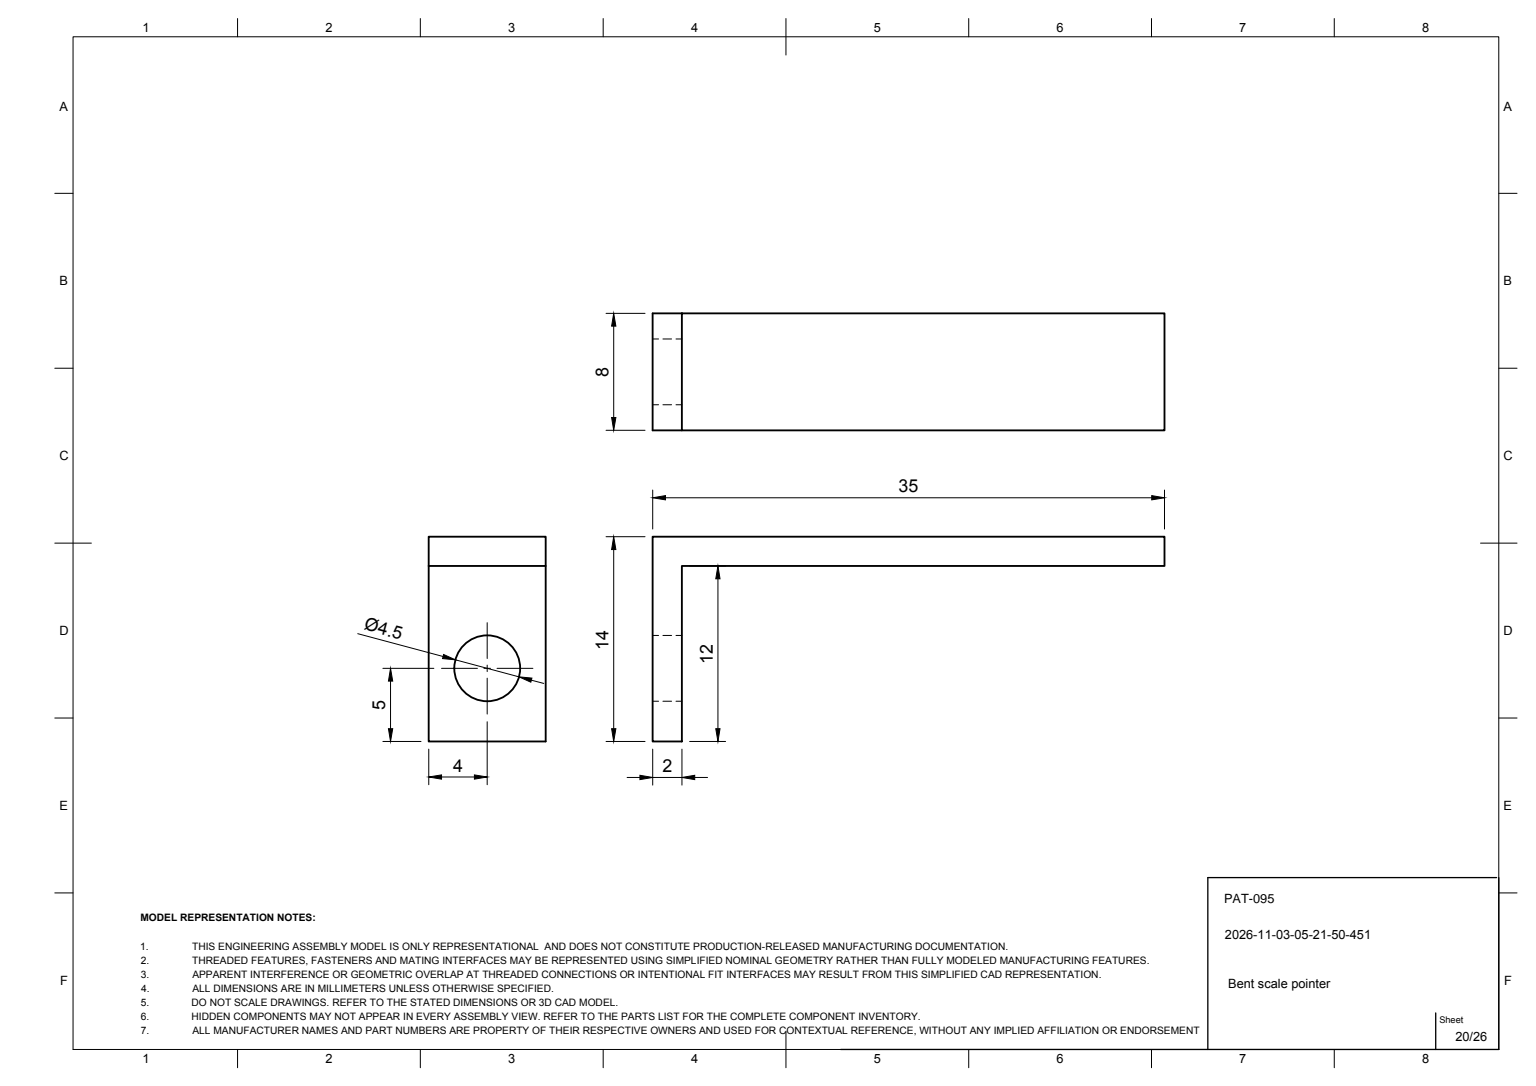
ISO-10303-21;
HEADER;
/* Generated by software containing ST-Developer
 * from STEP Tools, Inc. (www.steptools.com) 
 */

FILE_DESCRIPTION(
/* description */ ('Single-Axis Profile-Rail Linear Slide'),
/* implementation_level */ '2;1');

FILE_NAME(
/* name */ 'Bent scale pointer.step',
/* time_stamp */ '2026-10-27T10:47:43-07:00',
/* author */ (''),
/* organization */ (''),
/* preprocessor_version */ 'ST-DEVELOPER v20.2',
/* originating_system */ 'Autodesk Translation Framework v15.17.0.0',
/* authorisation */ '');

FILE_SCHEMA (('AUTOMOTIVE_DESIGN { 1 0 10303 214 3 1 1 }'));
ENDSEC;

DATA;
#10=MECHANICAL_DESIGN_GEOMETRIC_PRESENTATION_REPRESENTATION('',(#345),#14478);
#291=SHAPE_REPRESENTATION_RELATIONSHIP('SRR','None',#14622,#318);
#318=ADVANCED_BREP_SHAPE_REPRESENTATION('',(#370),#14466);
#345=STYLED_ITEM('',(#14845),#370);
#370=MANIFOLD_SOLID_BREP('Body1',#8607);
#451=FACE_BOUND('',#1705,.T.);
#452=FACE_BOUND('',#1710,.T.);
#753=PLANE('',#9375);
#754=PLANE('',#9376);
#755=PLANE('',#9377);
#756=PLANE('',#9378);
#757=PLANE('',#9379);
#758=PLANE('',#9380);
#759=PLANE('',#9381);
#760=PLANE('',#9382);
#1175=FACE_OUTER_BOUND('',#1703,.T.);
#1176=FACE_OUTER_BOUND('',#1704,.T.);
#1177=FACE_OUTER_BOUND('',#1706,.T.);
#1178=FACE_OUTER_BOUND('',#1707,.T.);
#1179=FACE_OUTER_BOUND('',#1708,.T.);
#1180=FACE_OUTER_BOUND('',#1709,.T.);
#1181=FACE_OUTER_BOUND('',#1711,.T.);
#1182=FACE_OUTER_BOUND('',#1712,.T.);
#1183=FACE_OUTER_BOUND('',#1713,.T.);
#1703=EDGE_LOOP('',(#7541,#7542,#7543,#7544));
#1704=EDGE_LOOP('',(#7545,#7546,#7547,#7548));
#1705=EDGE_LOOP('',(#7549));
#1706=EDGE_LOOP('',(#7550,#7551,#7552,#7553));
#1707=EDGE_LOOP('',(#7554,#7555,#7556,#7557));
#1708=EDGE_LOOP('',(#7558,#7559,#7560,#7561));
#1709=EDGE_LOOP('',(#7562,#7563,#7564,#7565));
#1710=EDGE_LOOP('',(#7566));
#1711=EDGE_LOOP('',(#7567,#7568,#7569,#7570));
#1712=EDGE_LOOP('',(#7571,#7572,#7573,#7574,#7575,#7576));
#1713=EDGE_LOOP('',(#7577,#7578,#7579,#7580,#7581,#7582));
#2606=LINE('',#13793,#3577);
#2607=LINE('',#13798,#3578);
#2608=LINE('',#13800,#3579);
#2609=LINE('',#13802,#3580);
#2610=LINE('',#13803,#3581);
#2611=LINE('',#13806,#3582);
#2612=LINE('',#13808,#3583);
#2613=LINE('',#13809,#3584);
#2614=LINE('',#13812,#3585);
#2615=LINE('',#13814,#3586);
#2616=LINE('',#13815,#3587);
#2617=LINE('',#13818,#3588);
#2618=LINE('',#13820,#3589);
#2619=LINE('',#13821,#3590);
#2620=LINE('',#13824,#3591);
#2621=LINE('',#13826,#3592);
#2622=LINE('',#13827,#3593);
#2623=LINE('',#13829,#3594);
#2624=LINE('',#13830,#3595);
#3577=VECTOR('',#11297,0.225);
#3578=VECTOR('',#11302,1.);
#3579=VECTOR('',#11303,1.);
#3580=VECTOR('',#11304,1.);
#3581=VECTOR('',#11305,1.);
#3582=VECTOR('',#11308,1.);
#3583=VECTOR('',#11309,1.);
#3584=VECTOR('',#11310,1.);
#3585=VECTOR('',#11313,1.);
#3586=VECTOR('',#11314,1.);
#3587=VECTOR('',#11315,1.);
#3588=VECTOR('',#11318,1.);
#3589=VECTOR('',#11319,1.);
#3590=VECTOR('',#11320,1.);
#3591=VECTOR('',#11323,1.);
#3592=VECTOR('',#11324,1.);
#3593=VECTOR('',#11325,1.);
#3594=VECTOR('',#11328,1.);
#3595=VECTOR('',#11329,1.);
#3878=CIRCLE('',#9373,0.225);
#3879=CIRCLE('',#9374,0.225);
#4512=VERTEX_POINT('',#13790);
#4513=VERTEX_POINT('',#13792);
#4514=VERTEX_POINT('',#13796);
#4515=VERTEX_POINT('',#13797);
#4516=VERTEX_POINT('',#13799);
#4517=VERTEX_POINT('',#13801);
#4518=VERTEX_POINT('',#13805);
#4519=VERTEX_POINT('',#13807);
#4520=VERTEX_POINT('',#13811);
#4521=VERTEX_POINT('',#13813);
#4522=VERTEX_POINT('',#13817);
#4523=VERTEX_POINT('',#13819);
#4524=VERTEX_POINT('',#13823);
#4525=VERTEX_POINT('',#13825);
#5548=EDGE_CURVE('',#4512,#4512,#3878,.T.);
#5549=EDGE_CURVE('',#4512,#4513,#2606,.T.);
#5550=EDGE_CURVE('',#4513,#4513,#3879,.T.);
#5551=EDGE_CURVE('',#4514,#4515,#2607,.T.);
#5552=EDGE_CURVE('',#4515,#4516,#2608,.T.);
#5553=EDGE_CURVE('',#4517,#4516,#2609,.T.);
#5554=EDGE_CURVE('',#4514,#4517,#2610,.T.);
#5555=EDGE_CURVE('',#4518,#4514,#2611,.T.);
#5556=EDGE_CURVE('',#4519,#4517,#2612,.T.);
#5557=EDGE_CURVE('',#4518,#4519,#2613,.T.);
#5558=EDGE_CURVE('',#4520,#4518,#2614,.T.);
#5559=EDGE_CURVE('',#4521,#4519,#2615,.T.);
#5560=EDGE_CURVE('',#4520,#4521,#2616,.T.);
#5561=EDGE_CURVE('',#4522,#4520,#2617,.T.);
#5562=EDGE_CURVE('',#4523,#4521,#2618,.T.);
#5563=EDGE_CURVE('',#4522,#4523,#2619,.T.);
#5564=EDGE_CURVE('',#4524,#4522,#2620,.T.);
#5565=EDGE_CURVE('',#4525,#4523,#2621,.T.);
#5566=EDGE_CURVE('',#4524,#4525,#2622,.T.);
#5567=EDGE_CURVE('',#4515,#4524,#2623,.T.);
#5568=EDGE_CURVE('',#4516,#4525,#2624,.T.);
#7541=ORIENTED_EDGE('',*,*,#5548,.F.);
#7542=ORIENTED_EDGE('',*,*,#5549,.T.);
#7543=ORIENTED_EDGE('',*,*,#5550,.F.);
#7544=ORIENTED_EDGE('',*,*,#5549,.F.);
#7545=ORIENTED_EDGE('',*,*,#5551,.T.);
#7546=ORIENTED_EDGE('',*,*,#5552,.T.);
#7547=ORIENTED_EDGE('',*,*,#5553,.F.);
#7548=ORIENTED_EDGE('',*,*,#5554,.F.);
#7549=ORIENTED_EDGE('',*,*,#5550,.T.);
#7550=ORIENTED_EDGE('',*,*,#5555,.T.);
#7551=ORIENTED_EDGE('',*,*,#5554,.T.);
#7552=ORIENTED_EDGE('',*,*,#5556,.F.);
#7553=ORIENTED_EDGE('',*,*,#5557,.F.);
#7554=ORIENTED_EDGE('',*,*,#5558,.T.);
#7555=ORIENTED_EDGE('',*,*,#5557,.T.);
#7556=ORIENTED_EDGE('',*,*,#5559,.F.);
#7557=ORIENTED_EDGE('',*,*,#5560,.F.);
#7558=ORIENTED_EDGE('',*,*,#5561,.T.);
#7559=ORIENTED_EDGE('',*,*,#5560,.T.);
#7560=ORIENTED_EDGE('',*,*,#5562,.F.);
#7561=ORIENTED_EDGE('',*,*,#5563,.F.);
#7562=ORIENTED_EDGE('',*,*,#5564,.T.);
#7563=ORIENTED_EDGE('',*,*,#5563,.T.);
#7564=ORIENTED_EDGE('',*,*,#5565,.F.);
#7565=ORIENTED_EDGE('',*,*,#5566,.F.);
#7566=ORIENTED_EDGE('',*,*,#5548,.T.);
#7567=ORIENTED_EDGE('',*,*,#5567,.T.);
#7568=ORIENTED_EDGE('',*,*,#5566,.T.);
#7569=ORIENTED_EDGE('',*,*,#5568,.F.);
#7570=ORIENTED_EDGE('',*,*,#5552,.F.);
#7571=ORIENTED_EDGE('',*,*,#5568,.T.);
#7572=ORIENTED_EDGE('',*,*,#5565,.T.);
#7573=ORIENTED_EDGE('',*,*,#5562,.T.);
#7574=ORIENTED_EDGE('',*,*,#5559,.T.);
#7575=ORIENTED_EDGE('',*,*,#5556,.T.);
#7576=ORIENTED_EDGE('',*,*,#5553,.T.);
#7577=ORIENTED_EDGE('',*,*,#5567,.F.);
#7578=ORIENTED_EDGE('',*,*,#5551,.F.);
#7579=ORIENTED_EDGE('',*,*,#5555,.F.);
#7580=ORIENTED_EDGE('',*,*,#5558,.F.);
#7581=ORIENTED_EDGE('',*,*,#5561,.F.);
#7582=ORIENTED_EDGE('',*,*,#5564,.F.);
#8115=CYLINDRICAL_SURFACE('',#9372,0.225);
#8469=ADVANCED_FACE('',(#1175),#8115,.F.);
#8470=ADVANCED_FACE('',(#1176,#451),#753,.T.);
#8471=ADVANCED_FACE('',(#1177),#754,.T.);
#8472=ADVANCED_FACE('',(#1178),#755,.T.);
#8473=ADVANCED_FACE('',(#1179),#756,.T.);
#8474=ADVANCED_FACE('',(#1180,#452),#757,.T.);
#8475=ADVANCED_FACE('',(#1181),#758,.T.);
#8476=ADVANCED_FACE('',(#1182),#759,.T.);
#8477=ADVANCED_FACE('',(#1183),#760,.F.);
#8607=CLOSED_SHELL('',(#8469,#8470,#8471,#8472,#8473,#8474,#8475,#8476,
#8477));
#9371=AXIS2_PLACEMENT_3D('',#13788,#11291,#11292);
#9372=AXIS2_PLACEMENT_3D('',#13789,#11293,#11294);
#9373=AXIS2_PLACEMENT_3D('',#13791,#11295,#11296);
#9374=AXIS2_PLACEMENT_3D('',#13794,#11298,#11299);
#9375=AXIS2_PLACEMENT_3D('',#13795,#11300,#11301);
#9376=AXIS2_PLACEMENT_3D('',#13804,#11306,#11307);
#9377=AXIS2_PLACEMENT_3D('',#13810,#11311,#11312);
#9378=AXIS2_PLACEMENT_3D('',#13816,#11316,#11317);
#9379=AXIS2_PLACEMENT_3D('',#13822,#11321,#11322);
#9380=AXIS2_PLACEMENT_3D('',#13828,#11326,#11327);
#9381=AXIS2_PLACEMENT_3D('',#13831,#11330,#11331);
#9382=AXIS2_PLACEMENT_3D('',#13832,#11332,#11333);
#11291=DIRECTION('axis',(0.,0.,1.));
#11292=DIRECTION('refdir',(1.,0.,0.));
#11293=DIRECTION('center_axis',(0.,0.,1.));
#11294=DIRECTION('ref_axis',(1.,0.,0.));
#11295=DIRECTION('center_axis',(0.,0.,1.));
#11296=DIRECTION('ref_axis',(1.,0.,0.));
#11297=DIRECTION('',(0.,0.,1.));
#11298=DIRECTION('center_axis',(0.,0.,-1.));
#11299=DIRECTION('ref_axis',(1.,0.,0.));
#11300=DIRECTION('center_axis',(0.,0.,1.));
#11301=DIRECTION('ref_axis',(0.,-1.,0.));
#11302=DIRECTION('',(0.,-1.,0.));
#11303=DIRECTION('',(1.,0.,0.));
#11304=DIRECTION('',(0.,-1.,0.));
#11305=DIRECTION('',(1.,0.,0.));
#11306=DIRECTION('center_axis',(0.,1.,0.));
#11307=DIRECTION('ref_axis',(0.,0.,1.));
#11308=DIRECTION('',(0.,0.,1.));
#11309=DIRECTION('',(0.,0.,1.));
#11310=DIRECTION('',(1.,0.,0.));
#11311=DIRECTION('center_axis',(0.,0.,-1.));
#11312=DIRECTION('ref_axis',(0.,1.,0.));
#11313=DIRECTION('',(0.,1.,0.));
#11314=DIRECTION('',(0.,1.,0.));
#11315=DIRECTION('',(1.,0.,0.));
#11316=DIRECTION('center_axis',(0.,-1.,0.));
#11317=DIRECTION('ref_axis',(0.,0.,-1.));
#11318=DIRECTION('',(0.,0.,-1.));
#11319=DIRECTION('',(0.,0.,-1.));
#11320=DIRECTION('',(1.,0.,0.));
#11321=DIRECTION('center_axis',(0.,0.,-1.));
#11322=DIRECTION('ref_axis',(0.,1.,0.));
#11323=DIRECTION('',(0.,1.,0.));
#11324=DIRECTION('',(0.,1.,0.));
#11325=DIRECTION('',(1.,0.,0.));
#11326=DIRECTION('center_axis',(0.,-1.,0.));
#11327=DIRECTION('ref_axis',(0.,0.,-1.));
#11328=DIRECTION('',(0.,0.,-1.));
#11329=DIRECTION('',(0.,0.,-1.));
#11330=DIRECTION('center_axis',(1.,0.,0.));
#11331=DIRECTION('ref_axis',(0.,0.,-1.));
#11332=DIRECTION('center_axis',(1.,0.,0.));
#11333=DIRECTION('ref_axis',(0.,0.,-1.));
#13788=CARTESIAN_POINT('',(0.,0.,0.));
#13789=CARTESIAN_POINT('Origin',(11.,3.5,6.3));
#13790=CARTESIAN_POINT('',(10.775,3.5,6.4));
#13791=CARTESIAN_POINT('Origin',(11.,3.5,6.4));
#13792=CARTESIAN_POINT('',(10.775,3.5,6.6));
#13793=CARTESIAN_POINT('',(10.775,3.5,6.3));
#13794=CARTESIAN_POINT('Origin',(11.,3.5,6.6));
#13795=CARTESIAN_POINT('Origin',(10.6,4.4,6.6));
#13796=CARTESIAN_POINT('',(10.6,4.4,6.6));
#13797=CARTESIAN_POINT('',(10.6,3.,6.6));
#13798=CARTESIAN_POINT('',(10.6,4.4,6.6));
#13799=CARTESIAN_POINT('',(11.4,3.,6.6));
#13800=CARTESIAN_POINT('',(10.6,3.,6.6));
#13801=CARTESIAN_POINT('',(11.4,4.4,6.6));
#13802=CARTESIAN_POINT('',(11.4,4.4,6.6));
#13803=CARTESIAN_POINT('',(10.6,4.4,6.6));
#13804=CARTESIAN_POINT('Origin',(10.6,4.4,3.1));
#13805=CARTESIAN_POINT('',(10.6,4.4,3.1));
#13806=CARTESIAN_POINT('',(10.6,4.4,3.1));
#13807=CARTESIAN_POINT('',(11.4,4.4,3.1));
#13808=CARTESIAN_POINT('',(11.4,4.4,3.1));
#13809=CARTESIAN_POINT('',(10.6,4.4,3.1));
#13810=CARTESIAN_POINT('Origin',(10.6,4.2,3.1));
#13811=CARTESIAN_POINT('',(10.6,4.2,3.1));
#13812=CARTESIAN_POINT('',(10.6,4.2,3.1));
#13813=CARTESIAN_POINT('',(11.4,4.2,3.1));
#13814=CARTESIAN_POINT('',(11.4,4.2,3.1));
#13815=CARTESIAN_POINT('',(10.6,4.2,3.1));
#13816=CARTESIAN_POINT('Origin',(10.6,4.2,6.4));
#13817=CARTESIAN_POINT('',(10.6,4.2,6.4));
#13818=CARTESIAN_POINT('',(10.6,4.2,6.4));
#13819=CARTESIAN_POINT('',(11.4,4.2,6.4));
#13820=CARTESIAN_POINT('',(11.4,4.2,6.4));
#13821=CARTESIAN_POINT('',(10.6,4.2,6.4));
#13822=CARTESIAN_POINT('Origin',(10.6,3.,6.4));
#13823=CARTESIAN_POINT('',(10.6,3.,6.4));
#13824=CARTESIAN_POINT('',(10.6,3.,6.4));
#13825=CARTESIAN_POINT('',(11.4,3.,6.4));
#13826=CARTESIAN_POINT('',(11.4,3.,6.4));
#13827=CARTESIAN_POINT('',(10.6,3.,6.4));
#13828=CARTESIAN_POINT('Origin',(10.6,3.,6.6));
#13829=CARTESIAN_POINT('',(10.6,3.,6.6));
#13830=CARTESIAN_POINT('',(11.4,3.,6.6));
#13831=CARTESIAN_POINT('Origin',(11.4,3.7,4.85));
#13832=CARTESIAN_POINT('Origin',(10.6,3.7,4.85));
#14434=UNCERTAINTY_MEASURE_WITH_UNIT(LENGTH_MEASURE(0.001),#14479,
'DISTANCE_ACCURACY_VALUE',
'Maximum model space distance between geometric entities at asserted c
onnectivities');
#14446=UNCERTAINTY_MEASURE_WITH_UNIT(LENGTH_MEASURE(0.001),#14479,
'DISTANCE_ACCURACY_VALUE',
'Maximum model space distance between geometric entities at asserted c
onnectivities');
#14466=(
GEOMETRIC_REPRESENTATION_CONTEXT(3)
GLOBAL_UNCERTAINTY_ASSIGNED_CONTEXT((#14434))
GLOBAL_UNIT_ASSIGNED_CONTEXT((#14479,#14481,#14482))
REPRESENTATION_CONTEXT('','3D')
);
#14478=(
GEOMETRIC_REPRESENTATION_CONTEXT(3)
GLOBAL_UNCERTAINTY_ASSIGNED_CONTEXT((#14446))
GLOBAL_UNIT_ASSIGNED_CONTEXT((#14479,#14481,#14482))
REPRESENTATION_CONTEXT('','3D')
);
#14479=(
LENGTH_UNIT()
NAMED_UNIT(*)
SI_UNIT(.CENTI.,.METRE.)
);
#14481=(
NAMED_UNIT(*)
PLANE_ANGLE_UNIT()
SI_UNIT($,.RADIAN.)
);
#14482=(
NAMED_UNIT(*)
SI_UNIT($,.STERADIAN.)
SOLID_ANGLE_UNIT()
);
#14502=SHAPE_DEFINITION_REPRESENTATION(#14533,#14622);
#14533=PRODUCT_DEFINITION_SHAPE('',$,#14654);
#14622=SHAPE_REPRESENTATION('',(#9371),#14466);
#14634=PRODUCT_DEFINITION_CONTEXT('part definition',#14729,'design');
#14654=PRODUCT_DEFINITION('Bent scale pointer','Bent scale pointer',#14685,
#14634);
#14685=PRODUCT_DEFINITION_FORMATION('',$,#14750);
#14729=APPLICATION_CONTEXT(
'Core Data for Automotive Mechanical Design Process');
#14730=PRODUCT_CONTEXT('part definition',#14729,'mechanical');
#14750=PRODUCT('Bent scale pointer','Bent scale pointer',
'Bent scale pointer',(#14730));
#14839=COLOUR_RGB('Off White',0.89,0.88,0.83);
#14840=FILL_AREA_STYLE_COLOUR('',#14839);
#14841=FILL_AREA_STYLE('',(#14840));
#14842=SURFACE_STYLE_FILL_AREA(#14841);
#14843=SURFACE_SIDE_STYLE('',(#14842));
#14844=SURFACE_STYLE_USAGE(.BOTH.,#14843);
#14845=PRESENTATION_STYLE_ASSIGNMENT((#14844));
ENDSEC;
END-ISO-10303-21;
